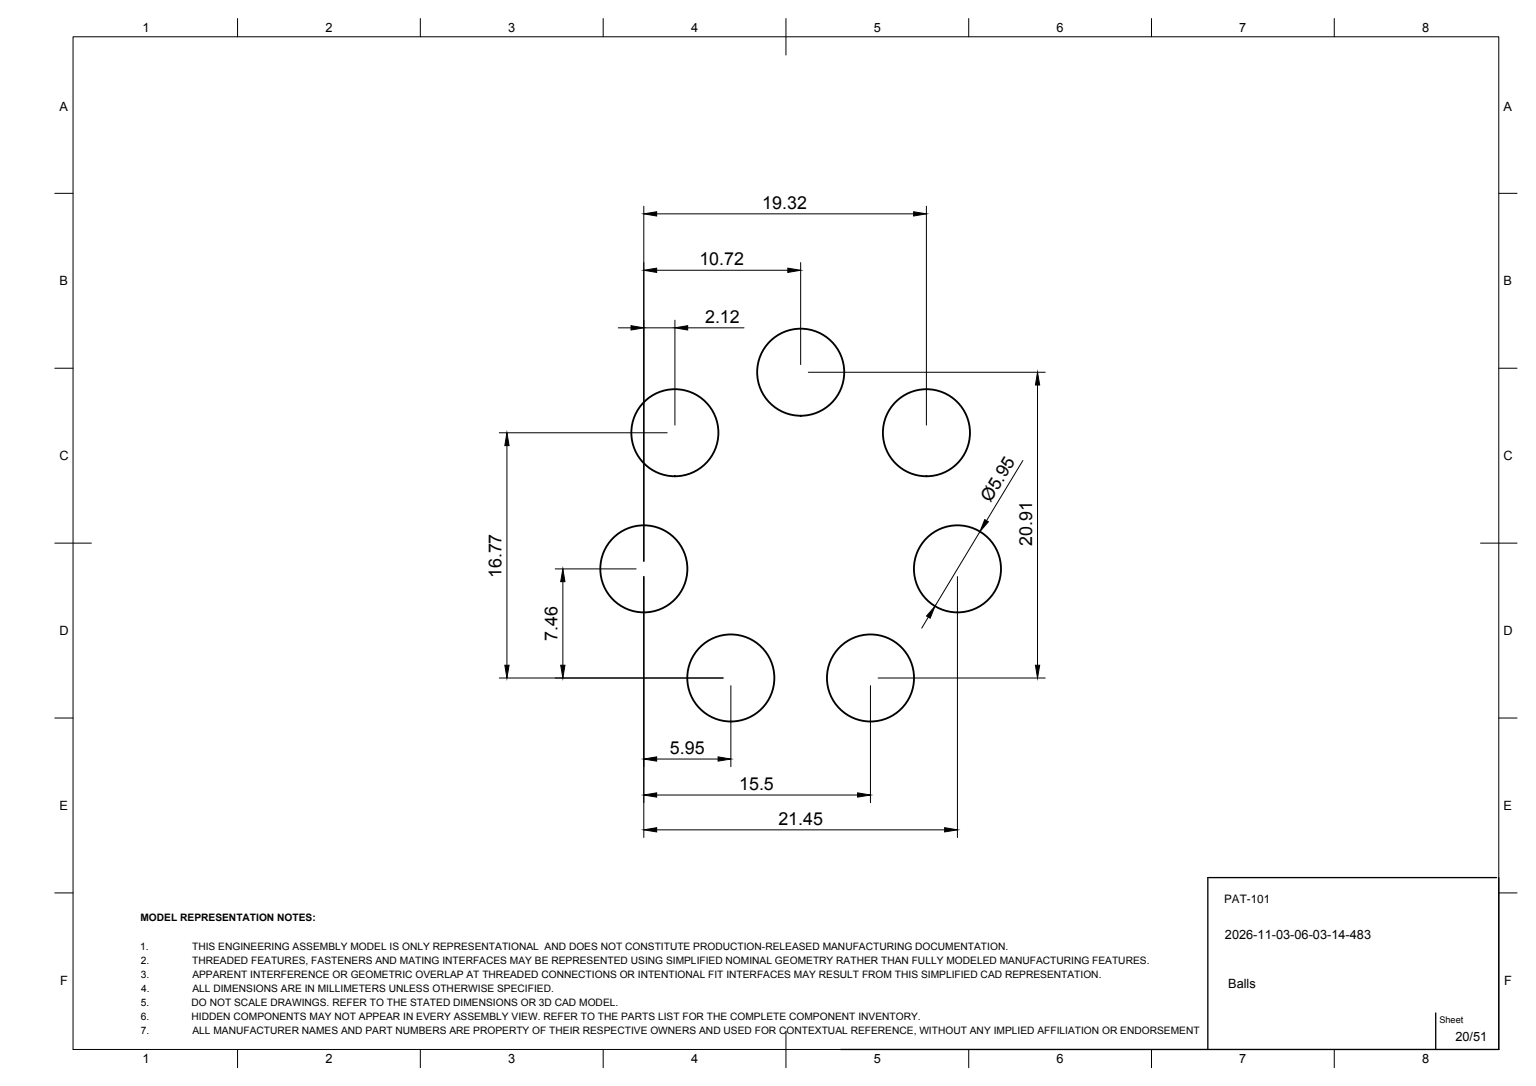
ISO-10303-21;
HEADER;
/* Generated by software containing ST-Developer
 * from STEP Tools, Inc. (www.steptools.com) 
 */

FILE_DESCRIPTION(
/* description */ ('Spur gear reduction stage 2-1 on bearing plates'),
/* implementation_level */ '2;1');

FILE_NAME(
/* name */ 'Balls.step',
/* time_stamp */ '2026-10-28T03:22:07-07:00',
/* author */ (''),
/* organization */ (''),
/* preprocessor_version */ 'ST-DEVELOPER v20.2',
/* originating_system */ 'Autodesk Translation Framework v15.17.0.0',
/* authorisation */ '');

FILE_SCHEMA (('AUTOMOTIVE_DESIGN { 1 0 10303 214 3 1 1 }'));
ENDSEC;

DATA;
#10=MECHANICAL_DESIGN_GEOMETRIC_PRESENTATION_REPRESENTATION('',(#962,#963,#964,#965,#966,#967,#968),#53909);
#795=SPHERICAL_SURFACE('',#12195,0.29765);
#796=SPHERICAL_SURFACE('',#12197,0.29765);
#797=SPHERICAL_SURFACE('',#12199,0.29765);
#798=SPHERICAL_SURFACE('',#12201,0.29765);
#799=SPHERICAL_SURFACE('',#12203,0.29765);
#800=SPHERICAL_SURFACE('',#12205,0.29765);
#801=SPHERICAL_SURFACE('',#12207,0.29765);
#876=SHAPE_REPRESENTATION_RELATIONSHIP('SRR','None',#54104,#919);
#919=ADVANCED_BREP_SHAPE_REPRESENTATION('',(#1018,#1019,#1020,#1021,#1022,
#1023,#1024),#53878);
#962=STYLED_ITEM('',(#54397),#1018);
#963=STYLED_ITEM('',(#54397),#1019);
#964=STYLED_ITEM('',(#54397),#1020);
#965=STYLED_ITEM('',(#54397),#1021);
#966=STYLED_ITEM('',(#54397),#1022);
#967=STYLED_ITEM('',(#54397),#1023);
#968=STYLED_ITEM('',(#54397),#1024);
#1018=MANIFOLD_SOLID_BREP('Body1',#11288);
#1019=MANIFOLD_SOLID_BREP('Body2',#11289);
#1020=MANIFOLD_SOLID_BREP('Body3',#11290);
#1021=MANIFOLD_SOLID_BREP('Body4',#11291);
#1022=MANIFOLD_SOLID_BREP('Body5',#11292);
#1023=MANIFOLD_SOLID_BREP('Body6',#11293);
#1024=MANIFOLD_SOLID_BREP('Body7',#11294);
#1683=FACE_OUTER_BOUND('',#2453,.T.);
#1684=FACE_OUTER_BOUND('',#2454,.T.);
#1685=FACE_OUTER_BOUND('',#2455,.T.);
#1686=FACE_OUTER_BOUND('',#2456,.T.);
#1687=FACE_OUTER_BOUND('',#2457,.T.);
#1688=FACE_OUTER_BOUND('',#2458,.T.);
#1689=FACE_OUTER_BOUND('',#2459,.T.);
#2453=EDGE_LOOP('',(#8072,#8073));
#2454=EDGE_LOOP('',(#8074,#8075));
#2455=EDGE_LOOP('',(#8076,#8077));
#2456=EDGE_LOOP('',(#8078,#8079));
#2457=EDGE_LOOP('',(#8080,#8081));
#2458=EDGE_LOOP('',(#8082,#8083));
#2459=EDGE_LOOP('',(#8084,#8085));
#4449=CIRCLE('',#12196,0.29765);
#4450=CIRCLE('',#12198,0.29765);
#4451=CIRCLE('',#12200,0.29765);
#4452=CIRCLE('',#12202,0.29765);
#4453=CIRCLE('',#12204,0.29765);
#4454=CIRCLE('',#12206,0.29765);
#4455=CIRCLE('',#12208,0.29765);
#5020=VERTEX_POINT('',#16771);
#5021=VERTEX_POINT('',#16772);
#5022=VERTEX_POINT('',#16775);
#5023=VERTEX_POINT('',#16776);
#5024=VERTEX_POINT('',#16779);
#5025=VERTEX_POINT('',#16780);
#5026=VERTEX_POINT('',#16783);
#5027=VERTEX_POINT('',#16784);
#5028=VERTEX_POINT('',#16787);
#5029=VERTEX_POINT('',#16788);
#5030=VERTEX_POINT('',#16791);
#5031=VERTEX_POINT('',#16792);
#5032=VERTEX_POINT('',#16795);
#5033=VERTEX_POINT('',#16796);
#6178=EDGE_CURVE('',#5020,#5021,#4449,.T.);
#6179=EDGE_CURVE('',#5022,#5023,#4450,.T.);
#6180=EDGE_CURVE('',#5024,#5025,#4451,.T.);
#6181=EDGE_CURVE('',#5026,#5027,#4452,.T.);
#6182=EDGE_CURVE('',#5028,#5029,#4453,.T.);
#6183=EDGE_CURVE('',#5030,#5031,#4454,.T.);
#6184=EDGE_CURVE('',#5032,#5033,#4455,.T.);
#8072=ORIENTED_EDGE('',*,*,#6178,.T.);
#8073=ORIENTED_EDGE('',*,*,#6178,.F.);
#8074=ORIENTED_EDGE('',*,*,#6179,.T.);
#8075=ORIENTED_EDGE('',*,*,#6179,.F.);
#8076=ORIENTED_EDGE('',*,*,#6180,.T.);
#8077=ORIENTED_EDGE('',*,*,#6180,.F.);
#8078=ORIENTED_EDGE('',*,*,#6181,.T.);
#8079=ORIENTED_EDGE('',*,*,#6181,.F.);
#8080=ORIENTED_EDGE('',*,*,#6182,.T.);
#8081=ORIENTED_EDGE('',*,*,#6182,.F.);
#8082=ORIENTED_EDGE('',*,*,#6183,.T.);
#8083=ORIENTED_EDGE('',*,*,#6183,.F.);
#8084=ORIENTED_EDGE('',*,*,#6184,.T.);
#8085=ORIENTED_EDGE('',*,*,#6184,.F.);
#10803=ADVANCED_FACE('',(#1683),#795,.T.);
#10804=ADVANCED_FACE('',(#1684),#796,.T.);
#10805=ADVANCED_FACE('',(#1685),#797,.T.);
#10806=ADVANCED_FACE('',(#1686),#798,.T.);
#10807=ADVANCED_FACE('',(#1687),#799,.T.);
#10808=ADVANCED_FACE('',(#1688),#800,.T.);
#10809=ADVANCED_FACE('',(#1689),#801,.T.);
#11288=CLOSED_SHELL('',(#10803));
#11289=CLOSED_SHELL('',(#10804));
#11290=CLOSED_SHELL('',(#10805));
#11291=CLOSED_SHELL('',(#10806));
#11292=CLOSED_SHELL('',(#10807));
#11293=CLOSED_SHELL('',(#10808));
#11294=CLOSED_SHELL('',(#10809));
#12194=AXIS2_PLACEMENT_3D('',#16769,#13928,#13929);
#12195=AXIS2_PLACEMENT_3D('',#16770,#13930,#13931);
#12196=AXIS2_PLACEMENT_3D('',#16773,#13932,#13933);
#12197=AXIS2_PLACEMENT_3D('',#16774,#13934,#13935);
#12198=AXIS2_PLACEMENT_3D('',#16777,#13936,#13937);
#12199=AXIS2_PLACEMENT_3D('',#16778,#13938,#13939);
#12200=AXIS2_PLACEMENT_3D('',#16781,#13940,#13941);
#12201=AXIS2_PLACEMENT_3D('',#16782,#13942,#13943);
#12202=AXIS2_PLACEMENT_3D('',#16785,#13944,#13945);
#12203=AXIS2_PLACEMENT_3D('',#16786,#13946,#13947);
#12204=AXIS2_PLACEMENT_3D('',#16789,#13948,#13949);
#12205=AXIS2_PLACEMENT_3D('',#16790,#13950,#13951);
#12206=AXIS2_PLACEMENT_3D('',#16793,#13952,#13953);
#12207=AXIS2_PLACEMENT_3D('',#16794,#13954,#13955);
#12208=AXIS2_PLACEMENT_3D('',#16797,#13956,#13957);
#13928=DIRECTION('axis',(0.,0.,1.));
#13929=DIRECTION('refdir',(1.,0.,0.));
#13930=DIRECTION('center_axis',(0.,0.,1.));
#13931=DIRECTION('ref_axis',(1.,0.,0.));
#13932=DIRECTION('center_axis',(1.22464679914735E-16,-1.,0.));
#13933=DIRECTION('ref_axis',(-1.,-1.22464679914735E-16,0.));
#13934=DIRECTION('center_axis',(0.78183148246803,0.,0.623489801858733));
#13935=DIRECTION('ref_axis',(0.623489801858734,0.,-0.78183148246803));
#13936=DIRECTION('center_axis',(7.63554790147315E-17,-1.,-9.57467422477103E-17));
#13937=DIRECTION('ref_axis',(-0.623489801858734,-1.22464679914735E-16,0.78183148246803));
#13938=DIRECTION('center_axis',(0.974927912181824,0.,-0.222520933956314));
#13939=DIRECTION('ref_axis',(-0.222520933956314,0.,-0.974927912181824));
#13940=DIRECTION('center_axis',(-2.7250954951288E-17,-1.,-1.19394234705288E-16));
#13941=DIRECTION('ref_axis',(0.222520933956314,-1.22464679914735E-16,0.974927912181824));
#13942=DIRECTION('center_axis',(0.433883739117558,0.,-0.900968867902419));
#13943=DIRECTION('ref_axis',(-0.900968867902419,0.,-0.433883739117558));
#13944=DIRECTION('center_axis',(-1.10336864020811E-16,-1.,-5.31354332312403E-17));
#13945=DIRECTION('ref_axis',(0.900968867902419,-1.22464679914735E-16,0.433883739117558));
#13946=DIRECTION('center_axis',(-0.433883739117558,0.,-0.900968867902419));
#13947=DIRECTION('ref_axis',(-0.900968867902419,0.,0.433883739117558));
#13948=DIRECTION('center_axis',(-1.10336864020811E-16,-1.,5.31354332312403E-17));
#13949=DIRECTION('ref_axis',(0.900968867902419,-1.22464679914735E-16,-0.433883739117558));
#13950=DIRECTION('center_axis',(-0.974927912181824,0.,-0.222520933956314));
#13951=DIRECTION('ref_axis',(-0.222520933956315,0.,0.974927912181824));
#13952=DIRECTION('center_axis',(-2.7250954951288E-17,-1.,1.19394234705288E-16));
#13953=DIRECTION('ref_axis',(0.222520933956315,-1.22464679914735E-16,-0.974927912181824));
#13954=DIRECTION('center_axis',(-0.78183148246803,0.,0.623489801858734));
#13955=DIRECTION('ref_axis',(0.623489801858733,0.,0.78183148246803));
#13956=DIRECTION('center_axis',(7.63554790147315E-17,-1.,9.57467422477103E-17));
#13957=DIRECTION('ref_axis',(-0.623489801858733,-1.22464679914735E-16,-0.78183148246803));
#16769=CARTESIAN_POINT('',(0.,0.,0.));
#16770=CARTESIAN_POINT('Origin',(1.1,0.,0.));
#16771=CARTESIAN_POINT('',(1.1,-2.23201749654651E-33,0.29765));
#16772=CARTESIAN_POINT('',(1.1,-2.23201749654651E-33,-0.29765));
#16773=CARTESIAN_POINT('Origin',(1.1,0.,0.));
#16774=CARTESIAN_POINT('Origin',(0.685838782044607,0.,-0.860014630714833));
#16775=CARTESIAN_POINT('',(0.918550922801216,-5.31350540756609E-33,-0.674432891191581));
#16776=CARTESIAN_POINT('',(0.453126641287998,8.49470414473068E-34,-1.04559637023808));
#16777=CARTESIAN_POINT('Origin',(0.685838782044607,0.,-0.860014630714833));
#16778=CARTESIAN_POINT('Origin',(-0.244773027351946,0.,-1.07242070340001));
#16779=CARTESIAN_POINT('',(0.0454142657089739,-2.23201749654651E-33,-1.1386540593921));
#16780=CARTESIAN_POINT('',(-0.534960320412865,-2.23201749654651E-33,-1.00618734740791));
#16781=CARTESIAN_POINT('Origin',(-0.244773027351946,0.,-1.07242070340001));
#16782=CARTESIAN_POINT('Origin',(-0.991065754692661,0.,-0.477272113029314));
#16783=CARTESIAN_POINT('',(-0.86192025974432,8.49470414473067E-34,-0.745445496560469));
#16784=CARTESIAN_POINT('',(-1.120211249641,-5.31350540756609E-33,-0.209098729498159));
#16785=CARTESIAN_POINT('Origin',(-0.991065754692661,0.,-0.477272113029314));
#16786=CARTESIAN_POINT('Origin',(-0.991065754692661,0.,0.477272113029314));
#16787=CARTESIAN_POINT('',(-1.120211249641,-2.23201749654651E-33,0.209098729498159));
#16788=CARTESIAN_POINT('',(-0.86192025974432,-2.23201749654651E-33,0.745445496560469));
#16789=CARTESIAN_POINT('Origin',(-0.991065754692661,0.,0.477272113029314));
#16790=CARTESIAN_POINT('Origin',(-0.244773027351946,0.,1.07242070340001));
#16791=CARTESIAN_POINT('',(-0.534960320412866,-2.23201749654651E-33,1.00618734740791));
#16792=CARTESIAN_POINT('',(0.0454142657089737,-2.23201749654651E-33,1.1386540593921));
#16793=CARTESIAN_POINT('Origin',(-0.244773027351946,0.,1.07242070340001));
#16794=CARTESIAN_POINT('Origin',(0.685838782044607,0.,0.860014630714833));
#16795=CARTESIAN_POINT('',(0.453126641287998,-2.23201749654651E-33,1.04559637023808));
#16796=CARTESIAN_POINT('',(0.918550922801216,-2.23201749654651E-33,0.674432891191581));
#16797=CARTESIAN_POINT('Origin',(0.685838782044607,0.,0.860014630714833));
#53828=UNCERTAINTY_MEASURE_WITH_UNIT(LENGTH_MEASURE(0.001),#53910,
'DISTANCE_ACCURACY_VALUE',
'Maximum model space distance between geometric entities at asserted c
onnectivities');
#53859=UNCERTAINTY_MEASURE_WITH_UNIT(LENGTH_MEASURE(0.001),#53910,
'DISTANCE_ACCURACY_VALUE',
'Maximum model space distance between geometric entities at asserted c
onnectivities');
#53878=(
GEOMETRIC_REPRESENTATION_CONTEXT(3)
GLOBAL_UNCERTAINTY_ASSIGNED_CONTEXT((#53828))
GLOBAL_UNIT_ASSIGNED_CONTEXT((#53910,#53912,#53913))
REPRESENTATION_CONTEXT('','3D')
);
#53909=(
GEOMETRIC_REPRESENTATION_CONTEXT(3)
GLOBAL_UNCERTAINTY_ASSIGNED_CONTEXT((#53859))
GLOBAL_UNIT_ASSIGNED_CONTEXT((#53910,#53912,#53913))
REPRESENTATION_CONTEXT('','3D')
);
#53910=(
LENGTH_UNIT()
NAMED_UNIT(*)
SI_UNIT(.CENTI.,.METRE.)
);
#53912=(
NAMED_UNIT(*)
PLANE_ANGLE_UNIT()
SI_UNIT($,.RADIAN.)
);
#53913=(
NAMED_UNIT(*)
SI_UNIT($,.STERADIAN.)
SOLID_ANGLE_UNIT()
);
#53932=SHAPE_DEFINITION_REPRESENTATION(#53981,#54104);
#53981=PRODUCT_DEFINITION_SHAPE('',$,#54154);
#54104=SHAPE_REPRESENTATION('',(#12194),#53878);
#54135=PRODUCT_DEFINITION_CONTEXT('part definition',#54284,'design');
#54154=PRODUCT_DEFINITION('Balls','Balls',#54203,#54135);
#54203=PRODUCT_DEFINITION_FORMATION('',$,#54304);
#54284=APPLICATION_CONTEXT(
'Core Data for Automotive Mechanical Design Process');
#54285=PRODUCT_CONTEXT('part definition',#54284,'mechanical');
#54304=PRODUCT('Balls','Balls','Balls',(#54285));
#54391=COLOUR_RGB('Grey',0.48,0.52,0.57);
#54392=FILL_AREA_STYLE_COLOUR('',#54391);
#54393=FILL_AREA_STYLE('',(#54392));
#54394=SURFACE_STYLE_FILL_AREA(#54393);
#54395=SURFACE_SIDE_STYLE('',(#54394));
#54396=SURFACE_STYLE_USAGE(.BOTH.,#54395);
#54397=PRESENTATION_STYLE_ASSIGNMENT((#54396));
ENDSEC;
END-ISO-10303-21;
